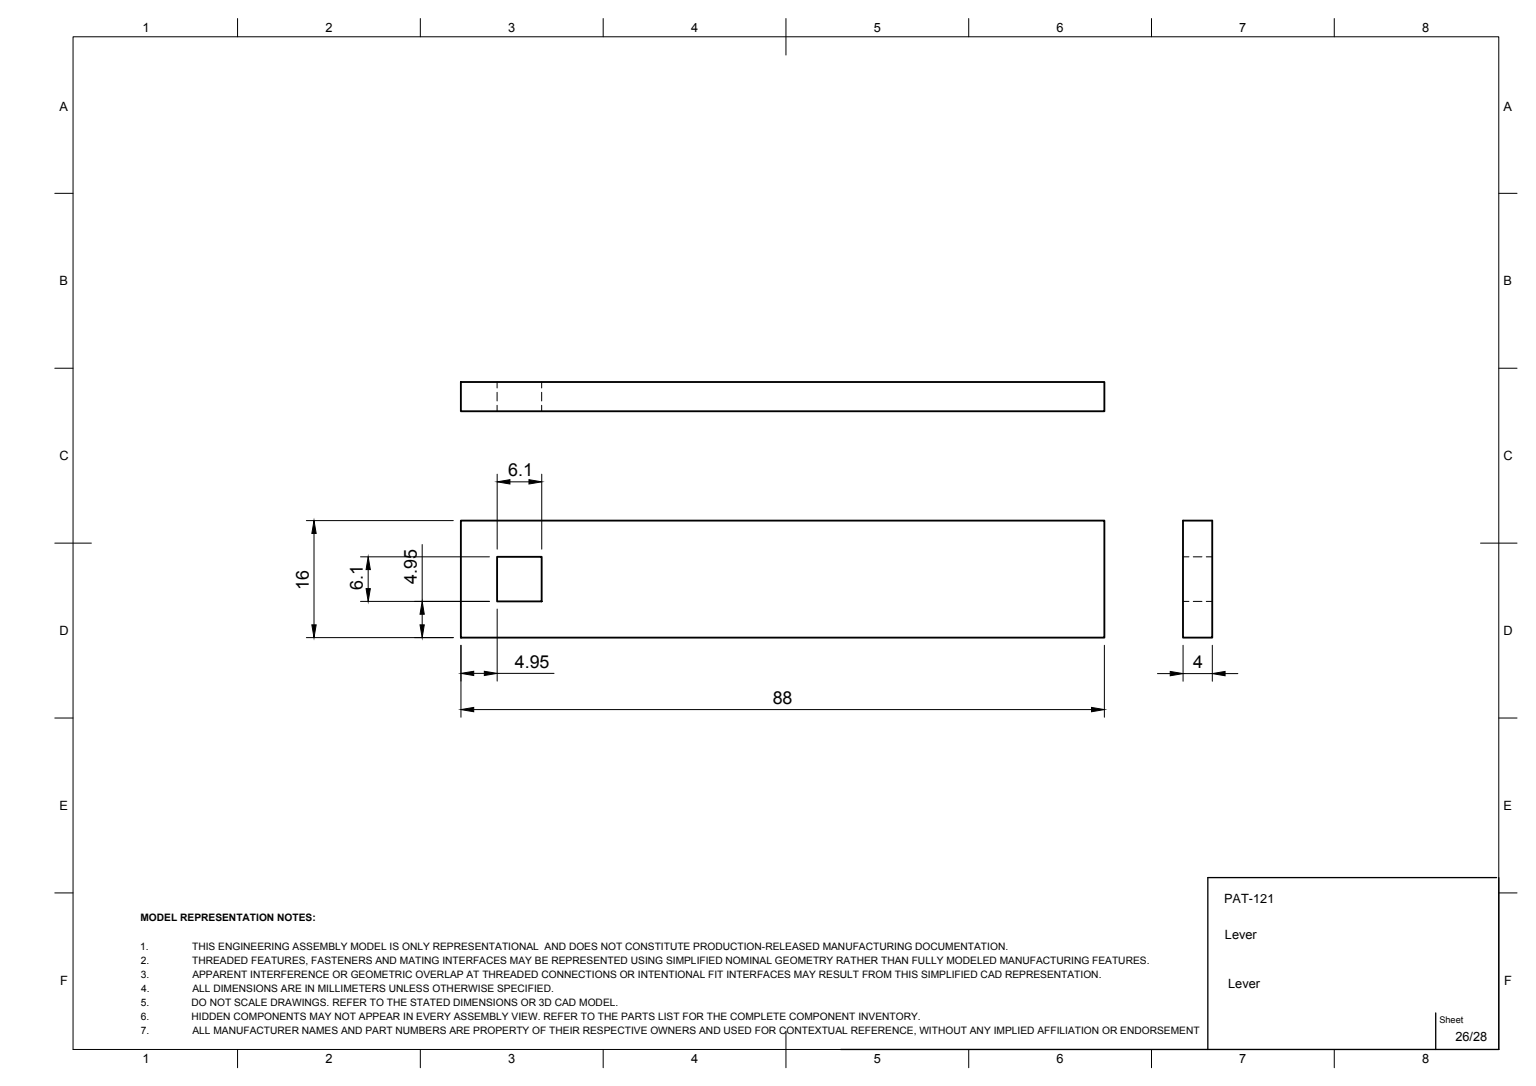
ISO-10303-21;
HEADER;
/* Generated by software containing ST-Developer
 * from STEP Tools, Inc. (www.steptools.com) 
 */

FILE_DESCRIPTION(
/* description */ ('Wall-mounted air drop station'),
/* implementation_level */ '2;1');

FILE_NAME(
/* name */ 'Lever.step',
/* time_stamp */ '2026-10-28T22:16:19-07:00',
/* author */ (''),
/* organization */ (''),
/* preprocessor_version */ 'ST-DEVELOPER v20.2',
/* originating_system */ 'Autodesk Translation Framework v15.17.0.0',
/* authorisation */ '');

FILE_SCHEMA (('AUTOMOTIVE_DESIGN { 1 0 10303 214 3 1 1 }'));
ENDSEC;

DATA;
#10=MECHANICAL_DESIGN_GEOMETRIC_PRESENTATION_REPRESENTATION('',(#369),#10517);
#311=SHAPE_REPRESENTATION_RELATIONSHIP('SRR','None',#10669,#340);
#340=ADVANCED_BREP_SHAPE_REPRESENTATION('',(#396),#10513);
#369=STYLED_ITEM('',(#10888),#396);
#396=MANIFOLD_SOLID_BREP('Body1',#5910);
#521=FACE_BOUND('',#1560,.T.);
#522=FACE_BOUND('',#1562,.T.);
#726=PLANE('',#6866);
#727=PLANE('',#6867);
#728=PLANE('',#6868);
#729=PLANE('',#6869);
#730=PLANE('',#6870);
#731=PLANE('',#6871);
#732=PLANE('',#6872);
#733=PLANE('',#6873);
#734=PLANE('',#6874);
#735=PLANE('',#6875);
#1074=FACE_OUTER_BOUND('',#1551,.T.);
#1075=FACE_OUTER_BOUND('',#1552,.T.);
#1076=FACE_OUTER_BOUND('',#1553,.T.);
#1077=FACE_OUTER_BOUND('',#1554,.T.);
#1078=FACE_OUTER_BOUND('',#1555,.T.);
#1079=FACE_OUTER_BOUND('',#1556,.T.);
#1080=FACE_OUTER_BOUND('',#1557,.T.);
#1081=FACE_OUTER_BOUND('',#1558,.T.);
#1082=FACE_OUTER_BOUND('',#1559,.T.);
#1083=FACE_OUTER_BOUND('',#1561,.T.);
#1551=EDGE_LOOP('',(#5287,#5288,#5289,#5290));
#1552=EDGE_LOOP('',(#5291,#5292,#5293,#5294));
#1553=EDGE_LOOP('',(#5295,#5296,#5297,#5298));
#1554=EDGE_LOOP('',(#5299,#5300,#5301,#5302));
#1555=EDGE_LOOP('',(#5303,#5304,#5305,#5306));
#1556=EDGE_LOOP('',(#5307,#5308,#5309,#5310));
#1557=EDGE_LOOP('',(#5311,#5312,#5313,#5314));
#1558=EDGE_LOOP('',(#5315,#5316,#5317,#5318));
#1559=EDGE_LOOP('',(#5319,#5320,#5321,#5322));
#1560=EDGE_LOOP('',(#5323,#5324,#5325,#5326));
#1561=EDGE_LOOP('',(#5327,#5328,#5329,#5330));
#1562=EDGE_LOOP('',(#5331,#5332,#5333,#5334));
#1995=LINE('',#10289,#2459);
#1996=LINE('',#10291,#2460);
#1997=LINE('',#10293,#2461);
#1998=LINE('',#10294,#2462);
#1999=LINE('',#10297,#2463);
#2000=LINE('',#10299,#2464);
#2001=LINE('',#10300,#2465);
#2002=LINE('',#10303,#2466);
#2003=LINE('',#10305,#2467);
#2004=LINE('',#10306,#2468);
#2005=LINE('',#10308,#2469);
#2006=LINE('',#10309,#2470);
#2007=LINE('',#10313,#2471);
#2008=LINE('',#10315,#2472);
#2009=LINE('',#10317,#2473);
#2010=LINE('',#10318,#2474);
#2011=LINE('',#10321,#2475);
#2012=LINE('',#10323,#2476);
#2013=LINE('',#10324,#2477);
#2014=LINE('',#10327,#2478);
#2015=LINE('',#10329,#2479);
#2016=LINE('',#10330,#2480);
#2017=LINE('',#10332,#2481);
#2018=LINE('',#10333,#2482);
#2459=VECTOR('',#8591,1.);
#2460=VECTOR('',#8592,1.);
#2461=VECTOR('',#8593,1.);
#2462=VECTOR('',#8594,1.);
#2463=VECTOR('',#8597,1.);
#2464=VECTOR('',#8598,1.);
#2465=VECTOR('',#8599,1.);
#2466=VECTOR('',#8602,1.);
#2467=VECTOR('',#8603,1.);
#2468=VECTOR('',#8604,1.);
#2469=VECTOR('',#8607,1.);
#2470=VECTOR('',#8608,1.);
#2471=VECTOR('',#8611,1.);
#2472=VECTOR('',#8612,1.);
#2473=VECTOR('',#8613,1.);
#2474=VECTOR('',#8614,1.);
#2475=VECTOR('',#8617,1.);
#2476=VECTOR('',#8618,1.);
#2477=VECTOR('',#8619,1.);
#2478=VECTOR('',#8622,1.);
#2479=VECTOR('',#8623,1.);
#2480=VECTOR('',#8624,1.);
#2481=VECTOR('',#8627,1.);
#2482=VECTOR('',#8628,1.);
#3197=VERTEX_POINT('',#10287);
#3198=VERTEX_POINT('',#10288);
#3199=VERTEX_POINT('',#10290);
#3200=VERTEX_POINT('',#10292);
#3201=VERTEX_POINT('',#10296);
#3202=VERTEX_POINT('',#10298);
#3203=VERTEX_POINT('',#10302);
#3204=VERTEX_POINT('',#10304);
#3205=VERTEX_POINT('',#10311);
#3206=VERTEX_POINT('',#10312);
#3207=VERTEX_POINT('',#10314);
#3208=VERTEX_POINT('',#10316);
#3209=VERTEX_POINT('',#10320);
#3210=VERTEX_POINT('',#10322);
#3211=VERTEX_POINT('',#10326);
#3212=VERTEX_POINT('',#10328);
#3901=EDGE_CURVE('',#3197,#3198,#1995,.T.);
#3902=EDGE_CURVE('',#3199,#3197,#1996,.T.);
#3903=EDGE_CURVE('',#3200,#3199,#1997,.T.);
#3904=EDGE_CURVE('',#3200,#3198,#1998,.T.);
#3905=EDGE_CURVE('',#3198,#3201,#1999,.T.);
#3906=EDGE_CURVE('',#3202,#3200,#2000,.T.);
#3907=EDGE_CURVE('',#3202,#3201,#2001,.T.);
#3908=EDGE_CURVE('',#3201,#3203,#2002,.T.);
#3909=EDGE_CURVE('',#3204,#3202,#2003,.T.);
#3910=EDGE_CURVE('',#3204,#3203,#2004,.T.);
#3911=EDGE_CURVE('',#3203,#3197,#2005,.T.);
#3912=EDGE_CURVE('',#3199,#3204,#2006,.T.);
#3913=EDGE_CURVE('',#3205,#3206,#2007,.T.);
#3914=EDGE_CURVE('',#3206,#3207,#2008,.T.);
#3915=EDGE_CURVE('',#3208,#3207,#2009,.T.);
#3916=EDGE_CURVE('',#3205,#3208,#2010,.T.);
#3917=EDGE_CURVE('',#3209,#3205,#2011,.T.);
#3918=EDGE_CURVE('',#3210,#3208,#2012,.T.);
#3919=EDGE_CURVE('',#3209,#3210,#2013,.T.);
#3920=EDGE_CURVE('',#3211,#3209,#2014,.T.);
#3921=EDGE_CURVE('',#3212,#3210,#2015,.T.);
#3922=EDGE_CURVE('',#3211,#3212,#2016,.T.);
#3923=EDGE_CURVE('',#3206,#3211,#2017,.T.);
#3924=EDGE_CURVE('',#3207,#3212,#2018,.T.);
#5287=ORIENTED_EDGE('',*,*,#3901,.F.);
#5288=ORIENTED_EDGE('',*,*,#3902,.F.);
#5289=ORIENTED_EDGE('',*,*,#3903,.F.);
#5290=ORIENTED_EDGE('',*,*,#3904,.T.);
#5291=ORIENTED_EDGE('',*,*,#3905,.F.);
#5292=ORIENTED_EDGE('',*,*,#3904,.F.);
#5293=ORIENTED_EDGE('',*,*,#3906,.F.);
#5294=ORIENTED_EDGE('',*,*,#3907,.T.);
#5295=ORIENTED_EDGE('',*,*,#3908,.F.);
#5296=ORIENTED_EDGE('',*,*,#3907,.F.);
#5297=ORIENTED_EDGE('',*,*,#3909,.F.);
#5298=ORIENTED_EDGE('',*,*,#3910,.T.);
#5299=ORIENTED_EDGE('',*,*,#3911,.F.);
#5300=ORIENTED_EDGE('',*,*,#3910,.F.);
#5301=ORIENTED_EDGE('',*,*,#3912,.F.);
#5302=ORIENTED_EDGE('',*,*,#3902,.T.);
#5303=ORIENTED_EDGE('',*,*,#3913,.T.);
#5304=ORIENTED_EDGE('',*,*,#3914,.T.);
#5305=ORIENTED_EDGE('',*,*,#3915,.F.);
#5306=ORIENTED_EDGE('',*,*,#3916,.F.);
#5307=ORIENTED_EDGE('',*,*,#3917,.T.);
#5308=ORIENTED_EDGE('',*,*,#3916,.T.);
#5309=ORIENTED_EDGE('',*,*,#3918,.F.);
#5310=ORIENTED_EDGE('',*,*,#3919,.F.);
#5311=ORIENTED_EDGE('',*,*,#3920,.T.);
#5312=ORIENTED_EDGE('',*,*,#3919,.T.);
#5313=ORIENTED_EDGE('',*,*,#3921,.F.);
#5314=ORIENTED_EDGE('',*,*,#3922,.F.);
#5315=ORIENTED_EDGE('',*,*,#3923,.T.);
#5316=ORIENTED_EDGE('',*,*,#3922,.T.);
#5317=ORIENTED_EDGE('',*,*,#3924,.F.);
#5318=ORIENTED_EDGE('',*,*,#3914,.F.);
#5319=ORIENTED_EDGE('',*,*,#3924,.T.);
#5320=ORIENTED_EDGE('',*,*,#3921,.T.);
#5321=ORIENTED_EDGE('',*,*,#3918,.T.);
#5322=ORIENTED_EDGE('',*,*,#3915,.T.);
#5323=ORIENTED_EDGE('',*,*,#3908,.T.);
#5324=ORIENTED_EDGE('',*,*,#3911,.T.);
#5325=ORIENTED_EDGE('',*,*,#3901,.T.);
#5326=ORIENTED_EDGE('',*,*,#3905,.T.);
#5327=ORIENTED_EDGE('',*,*,#3923,.F.);
#5328=ORIENTED_EDGE('',*,*,#3913,.F.);
#5329=ORIENTED_EDGE('',*,*,#3917,.F.);
#5330=ORIENTED_EDGE('',*,*,#3920,.F.);
#5331=ORIENTED_EDGE('',*,*,#3909,.T.);
#5332=ORIENTED_EDGE('',*,*,#3906,.T.);
#5333=ORIENTED_EDGE('',*,*,#3903,.T.);
#5334=ORIENTED_EDGE('',*,*,#3912,.T.);
#5847=ADVANCED_FACE('',(#1074),#726,.F.);
#5848=ADVANCED_FACE('',(#1075),#727,.F.);
#5849=ADVANCED_FACE('',(#1076),#728,.F.);
#5850=ADVANCED_FACE('',(#1077),#729,.F.);
#5851=ADVANCED_FACE('',(#1078),#730,.T.);
#5852=ADVANCED_FACE('',(#1079),#731,.T.);
#5853=ADVANCED_FACE('',(#1080),#732,.T.);
#5854=ADVANCED_FACE('',(#1081),#733,.T.);
#5855=ADVANCED_FACE('',(#1082,#521),#734,.T.);
#5856=ADVANCED_FACE('',(#1083,#522),#735,.F.);
#5910=CLOSED_SHELL('',(#5847,#5848,#5849,#5850,#5851,#5852,#5853,#5854,
#5855,#5856));
#6865=AXIS2_PLACEMENT_3D('',#10285,#8587,#8588);
#6866=AXIS2_PLACEMENT_3D('',#10286,#8589,#8590);
#6867=AXIS2_PLACEMENT_3D('',#10295,#8595,#8596);
#6868=AXIS2_PLACEMENT_3D('',#10301,#8600,#8601);
#6869=AXIS2_PLACEMENT_3D('',#10307,#8605,#8606);
#6870=AXIS2_PLACEMENT_3D('',#10310,#8609,#8610);
#6871=AXIS2_PLACEMENT_3D('',#10319,#8615,#8616);
#6872=AXIS2_PLACEMENT_3D('',#10325,#8620,#8621);
#6873=AXIS2_PLACEMENT_3D('',#10331,#8625,#8626);
#6874=AXIS2_PLACEMENT_3D('',#10334,#8629,#8630);
#6875=AXIS2_PLACEMENT_3D('',#10335,#8631,#8632);
#8587=DIRECTION('axis',(0.,0.,1.));
#8588=DIRECTION('refdir',(1.,0.,0.));
#8589=DIRECTION('center_axis',(0.,-1.,0.));
#8590=DIRECTION('ref_axis',(1.,0.,0.));
#8591=DIRECTION('',(-1.,0.,0.));
#8592=DIRECTION('',(0.,0.,1.));
#8593=DIRECTION('',(1.,0.,0.));
#8594=DIRECTION('',(0.,0.,1.));
#8595=DIRECTION('center_axis',(-1.,0.,0.));
#8596=DIRECTION('ref_axis',(0.,-1.,0.));
#8597=DIRECTION('',(0.,1.,0.));
#8598=DIRECTION('',(0.,-1.,0.));
#8599=DIRECTION('',(0.,0.,1.));
#8600=DIRECTION('center_axis',(0.,1.,0.));
#8601=DIRECTION('ref_axis',(-1.,0.,0.));
#8602=DIRECTION('',(1.,0.,0.));
#8603=DIRECTION('',(-1.,0.,0.));
#8604=DIRECTION('',(0.,0.,1.));
#8605=DIRECTION('center_axis',(1.,0.,0.));
#8606=DIRECTION('ref_axis',(0.,1.,0.));
#8607=DIRECTION('',(0.,-1.,0.));
#8608=DIRECTION('',(0.,1.,0.));
#8609=DIRECTION('center_axis',(0.,1.,0.));
#8610=DIRECTION('ref_axis',(-1.,0.,0.));
#8611=DIRECTION('',(-1.,0.,0.));
#8612=DIRECTION('',(0.,0.,1.));
#8613=DIRECTION('',(-1.,0.,0.));
#8614=DIRECTION('',(0.,0.,1.));
#8615=DIRECTION('center_axis',(1.,0.,0.));
#8616=DIRECTION('ref_axis',(0.,1.,0.));
#8617=DIRECTION('',(0.,1.,0.));
#8618=DIRECTION('',(0.,1.,0.));
#8619=DIRECTION('',(0.,0.,1.));
#8620=DIRECTION('center_axis',(0.,-1.,0.));
#8621=DIRECTION('ref_axis',(1.,0.,0.));
#8622=DIRECTION('',(1.,0.,0.));
#8623=DIRECTION('',(1.,0.,0.));
#8624=DIRECTION('',(0.,0.,1.));
#8625=DIRECTION('center_axis',(-1.,0.,0.));
#8626=DIRECTION('ref_axis',(0.,-1.,0.));
#8627=DIRECTION('',(0.,-1.,0.));
#8628=DIRECTION('',(0.,-1.,0.));
#8629=DIRECTION('center_axis',(0.,0.,1.));
#8630=DIRECTION('ref_axis',(1.,0.,0.));
#8631=DIRECTION('center_axis',(0.,0.,1.));
#8632=DIRECTION('ref_axis',(1.,0.,0.));
#10285=CARTESIAN_POINT('',(0.,0.,0.));
#10286=CARTESIAN_POINT('Origin',(-0.305,-0.305,8.9));
#10287=CARTESIAN_POINT('',(0.305,-0.305,9.4));
#10288=CARTESIAN_POINT('',(-0.305,-0.305,9.4));
#10289=CARTESIAN_POINT('',(1.6475,-0.305,9.4));
#10290=CARTESIAN_POINT('',(0.305,-0.305,9.));
#10291=CARTESIAN_POINT('',(0.305,-0.305,8.9));
#10292=CARTESIAN_POINT('',(-0.305,-0.305,9.));
#10293=CARTESIAN_POINT('',(1.6475,-0.305,9.));
#10294=CARTESIAN_POINT('',(-0.305,-0.305,8.9));
#10295=CARTESIAN_POINT('Origin',(-0.305,0.305,8.9));
#10296=CARTESIAN_POINT('',(-0.305,0.305,9.4));
#10297=CARTESIAN_POINT('',(-0.305,0.1525,9.4));
#10298=CARTESIAN_POINT('',(-0.305,0.305,9.));
#10299=CARTESIAN_POINT('',(-0.305,0.1525,9.));
#10300=CARTESIAN_POINT('',(-0.305,0.305,8.9));
#10301=CARTESIAN_POINT('Origin',(0.305,0.305,8.9));
#10302=CARTESIAN_POINT('',(0.305,0.305,9.4));
#10303=CARTESIAN_POINT('',(1.9525,0.305,9.4));
#10304=CARTESIAN_POINT('',(0.305,0.305,9.));
#10305=CARTESIAN_POINT('',(1.9525,0.305,9.));
#10306=CARTESIAN_POINT('',(0.305,0.305,8.9));
#10307=CARTESIAN_POINT('Origin',(0.305,-0.305,8.9));
#10308=CARTESIAN_POINT('',(0.305,-0.1525,9.4));
#10309=CARTESIAN_POINT('',(0.305,-0.1525,9.));
#10310=CARTESIAN_POINT('Origin',(8.,0.8,9.));
#10311=CARTESIAN_POINT('',(8.,0.8,9.));
#10312=CARTESIAN_POINT('',(-0.8,0.8,9.));
#10313=CARTESIAN_POINT('',(8.,0.8,9.));
#10314=CARTESIAN_POINT('',(-0.8,0.8,9.4));
#10315=CARTESIAN_POINT('',(-0.8,0.8,9.));
#10316=CARTESIAN_POINT('',(8.,0.8,9.4));
#10317=CARTESIAN_POINT('',(8.,0.8,9.4));
#10318=CARTESIAN_POINT('',(8.,0.8,9.));
#10319=CARTESIAN_POINT('Origin',(8.,-0.8,9.));
#10320=CARTESIAN_POINT('',(8.,-0.8,9.));
#10321=CARTESIAN_POINT('',(8.,-0.8,9.));
#10322=CARTESIAN_POINT('',(8.,-0.8,9.4));
#10323=CARTESIAN_POINT('',(8.,-0.8,9.4));
#10324=CARTESIAN_POINT('',(8.,-0.8,9.));
#10325=CARTESIAN_POINT('Origin',(-0.8,-0.8,9.));
#10326=CARTESIAN_POINT('',(-0.8,-0.8,9.));
#10327=CARTESIAN_POINT('',(-0.8,-0.8,9.));
#10328=CARTESIAN_POINT('',(-0.8,-0.8,9.4));
#10329=CARTESIAN_POINT('',(-0.8,-0.8,9.4));
#10330=CARTESIAN_POINT('',(-0.8,-0.8,9.));
#10331=CARTESIAN_POINT('Origin',(-0.8,0.8,9.));
#10332=CARTESIAN_POINT('',(-0.8,0.8,9.));
#10333=CARTESIAN_POINT('',(-0.8,0.8,9.4));
#10334=CARTESIAN_POINT('Origin',(3.6,0.,9.4));
#10335=CARTESIAN_POINT('Origin',(3.6,0.,9.));
#10480=UNCERTAINTY_MEASURE_WITH_UNIT(LENGTH_MEASURE(0.001),#10518,
'DISTANCE_ACCURACY_VALUE',
'Maximum model space distance between geometric entities at asserted c
onnectivities');
#10484=UNCERTAINTY_MEASURE_WITH_UNIT(LENGTH_MEASURE(0.001),#10518,
'DISTANCE_ACCURACY_VALUE',
'Maximum model space distance between geometric entities at asserted c
onnectivities');
#10513=(
GEOMETRIC_REPRESENTATION_CONTEXT(3)
GLOBAL_UNCERTAINTY_ASSIGNED_CONTEXT((#10480))
GLOBAL_UNIT_ASSIGNED_CONTEXT((#10518,#10520,#10521))
REPRESENTATION_CONTEXT('','3D')
);
#10517=(
GEOMETRIC_REPRESENTATION_CONTEXT(3)
GLOBAL_UNCERTAINTY_ASSIGNED_CONTEXT((#10484))
GLOBAL_UNIT_ASSIGNED_CONTEXT((#10518,#10520,#10521))
REPRESENTATION_CONTEXT('','3D')
);
#10518=(
LENGTH_UNIT()
NAMED_UNIT(*)
SI_UNIT(.CENTI.,.METRE.)
);
#10520=(
NAMED_UNIT(*)
PLANE_ANGLE_UNIT()
SI_UNIT($,.RADIAN.)
);
#10521=(
NAMED_UNIT(*)
SI_UNIT($,.STERADIAN.)
SOLID_ANGLE_UNIT()
);
#10550=SHAPE_DEFINITION_REPRESENTATION(#10629,#10669);
#10629=PRODUCT_DEFINITION_SHAPE('',$,#10702);
#10669=SHAPE_REPRESENTATION('',(#6865),#10513);
#10673=PRODUCT_DEFINITION_CONTEXT('part definition',#10771,'design');
#10702=PRODUCT_DEFINITION('Lever','Lever',#10734,#10673);
#10734=PRODUCT_DEFINITION_FORMATION('',$,#10801);
#10771=APPLICATION_CONTEXT(
'Core Data for Automotive Mechanical Design Process');
#10772=PRODUCT_CONTEXT('part definition',#10771,'mechanical');
#10801=PRODUCT('Lever','Lever','Lever',(#10772));
#10882=COLOUR_RGB('Off White',0.89,0.88,0.83);
#10883=FILL_AREA_STYLE_COLOUR('',#10882);
#10884=FILL_AREA_STYLE('',(#10883));
#10885=SURFACE_STYLE_FILL_AREA(#10884);
#10886=SURFACE_SIDE_STYLE('',(#10885));
#10887=SURFACE_STYLE_USAGE(.BOTH.,#10886);
#10888=PRESENTATION_STYLE_ASSIGNMENT((#10887));
ENDSEC;
END-ISO-10303-21;
